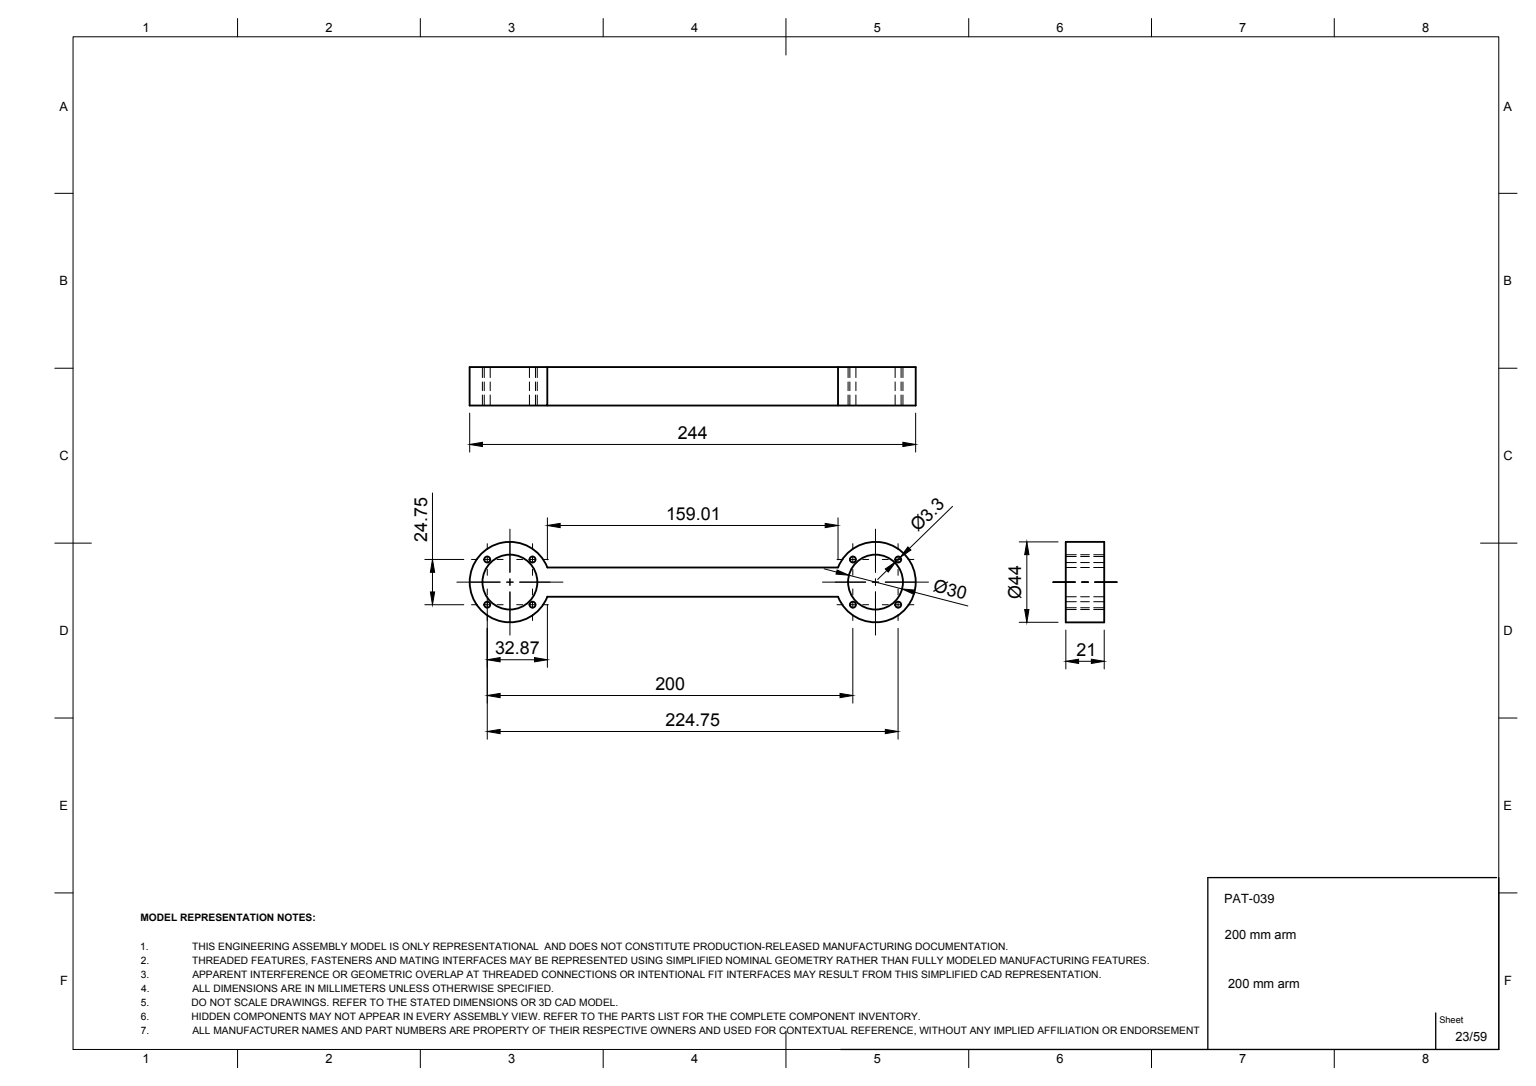
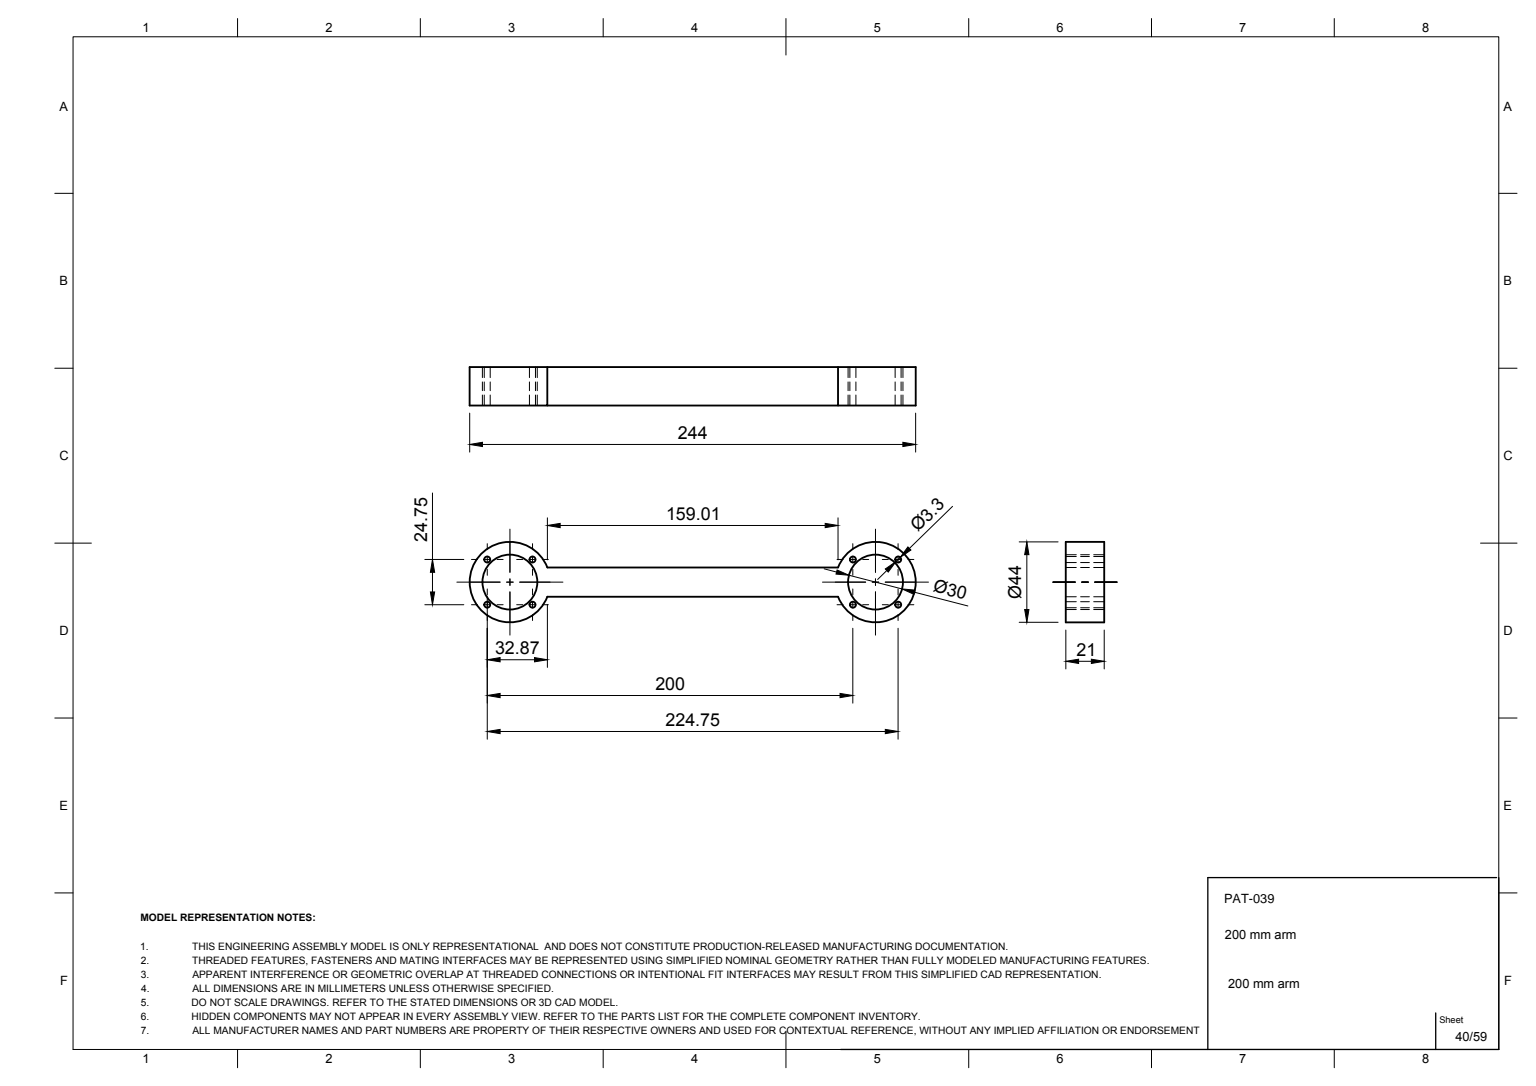
ISO-10303-21;
HEADER;
/* Generated by software containing ST-Developer
 * from STEP Tools, Inc. (www.steptools.com) 
 */

FILE_DESCRIPTION(
/* description */ ('Four-bar parallelogram arm'),
/* implementation_level */ '2;1');

FILE_NAME(
/* name */ '200 mm arm.step',
/* time_stamp */ '2026-10-28T03:24:55-07:00',
/* author */ (''),
/* organization */ (''),
/* preprocessor_version */ 'ST-DEVELOPER v20.2',
/* originating_system */ 'Autodesk Translation Framework v15.17.0.0',
/* authorisation */ '');

FILE_SCHEMA (('AUTOMOTIVE_DESIGN { 1 0 10303 214 3 1 1 }'));
ENDSEC;

DATA;
#10=MECHANICAL_DESIGN_GEOMETRIC_PRESENTATION_REPRESENTATION('',(#639),#14512);
#539=SHAPE_REPRESENTATION_RELATIONSHIP('SRR','None',#14761,#589);
#589=ADVANCED_BREP_SHAPE_REPRESENTATION('',(#696),#14476);
#639=STYLED_ITEM('',(#15101),#696);
#696=MANIFOLD_SOLID_BREP('Body1',#7344);
#807=FACE_BOUND('',#1846,.T.);
#808=FACE_BOUND('',#1847,.T.);
#809=FACE_BOUND('',#1848,.T.);
#810=FACE_BOUND('',#1849,.T.);
#811=FACE_BOUND('',#1850,.T.);
#812=FACE_BOUND('',#1851,.T.);
#813=FACE_BOUND('',#1852,.T.);
#814=FACE_BOUND('',#1853,.T.);
#815=FACE_BOUND('',#1854,.T.);
#816=FACE_BOUND('',#1855,.T.);
#817=FACE_BOUND('',#1859,.T.);
#818=FACE_BOUND('',#1860,.T.);
#819=FACE_BOUND('',#1861,.T.);
#820=FACE_BOUND('',#1862,.T.);
#821=FACE_BOUND('',#1863,.T.);
#822=FACE_BOUND('',#1864,.T.);
#823=FACE_BOUND('',#1865,.T.);
#824=FACE_BOUND('',#1866,.T.);
#825=FACE_BOUND('',#1867,.T.);
#826=FACE_BOUND('',#1868,.T.);
#1089=PLANE('',#8243);
#1090=PLANE('',#8244);
#1091=PLANE('',#8246);
#1092=PLANE('',#8249);
#1341=FACE_OUTER_BOUND('',#1833,.T.);
#1342=FACE_OUTER_BOUND('',#1834,.T.);
#1343=FACE_OUTER_BOUND('',#1835,.T.);
#1344=FACE_OUTER_BOUND('',#1836,.T.);
#1345=FACE_OUTER_BOUND('',#1837,.T.);
#1346=FACE_OUTER_BOUND('',#1838,.T.);
#1347=FACE_OUTER_BOUND('',#1839,.T.);
#1348=FACE_OUTER_BOUND('',#1840,.T.);
#1349=FACE_OUTER_BOUND('',#1841,.T.);
#1350=FACE_OUTER_BOUND('',#1842,.T.);
#1351=FACE_OUTER_BOUND('',#1843,.T.);
#1352=FACE_OUTER_BOUND('',#1844,.T.);
#1353=FACE_OUTER_BOUND('',#1845,.T.);
#1354=FACE_OUTER_BOUND('',#1856,.T.);
#1355=FACE_OUTER_BOUND('',#1857,.T.);
#1356=FACE_OUTER_BOUND('',#1858,.T.);
#1833=EDGE_LOOP('',(#5550,#5551,#5552,#5553));
#1834=EDGE_LOOP('',(#5554,#5555,#5556,#5557));
#1835=EDGE_LOOP('',(#5558,#5559,#5560,#5561));
#1836=EDGE_LOOP('',(#5562,#5563,#5564,#5565));
#1837=EDGE_LOOP('',(#5566,#5567,#5568,#5569));
#1838=EDGE_LOOP('',(#5570,#5571,#5572,#5573));
#1839=EDGE_LOOP('',(#5574,#5575,#5576,#5577));
#1840=EDGE_LOOP('',(#5578,#5579,#5580,#5581));
#1841=EDGE_LOOP('',(#5582,#5583,#5584,#5585));
#1842=EDGE_LOOP('',(#5586,#5587,#5588,#5589));
#1843=EDGE_LOOP('',(#5590,#5591,#5592,#5593));
#1844=EDGE_LOOP('',(#5594,#5595,#5596,#5597));
#1845=EDGE_LOOP('',(#5598,#5599,#5600,#5601));
#1846=EDGE_LOOP('',(#5602));
#1847=EDGE_LOOP('',(#5603));
#1848=EDGE_LOOP('',(#5604));
#1849=EDGE_LOOP('',(#5605));
#1850=EDGE_LOOP('',(#5606));
#1851=EDGE_LOOP('',(#5607));
#1852=EDGE_LOOP('',(#5608));
#1853=EDGE_LOOP('',(#5609));
#1854=EDGE_LOOP('',(#5610));
#1855=EDGE_LOOP('',(#5611));
#1856=EDGE_LOOP('',(#5612,#5613,#5614,#5615));
#1857=EDGE_LOOP('',(#5616,#5617,#5618,#5619));
#1858=EDGE_LOOP('',(#5620,#5621,#5622,#5623));
#1859=EDGE_LOOP('',(#5624));
#1860=EDGE_LOOP('',(#5625));
#1861=EDGE_LOOP('',(#5626));
#1862=EDGE_LOOP('',(#5627));
#1863=EDGE_LOOP('',(#5628));
#1864=EDGE_LOOP('',(#5629));
#1865=EDGE_LOOP('',(#5630));
#1866=EDGE_LOOP('',(#5631));
#1867=EDGE_LOOP('',(#5632));
#1868=EDGE_LOOP('',(#5633));
#2475=LINE('',#12661,#2869);
#2476=LINE('',#12667,#2870);
#2477=LINE('',#12673,#2871);
#2478=LINE('',#12679,#2872);
#2479=LINE('',#12685,#2873);
#2480=LINE('',#12691,#2874);
#2481=LINE('',#12697,#2875);
#2482=LINE('',#12703,#2876);
#2483=LINE('',#12709,#2877);
#2484=LINE('',#12715,#2878);
#2485=LINE('',#12720,#2879);
#2486=LINE('',#12724,#2880);
#2487=LINE('',#12728,#2881);
#2488=LINE('',#12730,#2882);
#2489=LINE('',#12731,#2883);
#2490=LINE('',#12734,#2884);
#2491=LINE('',#12738,#2885);
#2492=LINE('',#12739,#2886);
#2869=VECTOR('',#9681,0.164999999999999);
#2870=VECTOR('',#9688,0.164999999999999);
#2871=VECTOR('',#9695,0.164999999999999);
#2872=VECTOR('',#9702,0.164999999999999);
#2873=VECTOR('',#9709,0.165);
#2874=VECTOR('',#9716,0.165);
#2875=VECTOR('',#9723,0.165);
#2876=VECTOR('',#9730,0.165);
#2877=VECTOR('',#9737,1.5);
#2878=VECTOR('',#9744,1.5);
#2879=VECTOR('',#9749,1.);
#2880=VECTOR('',#9752,1.);
#2881=VECTOR('',#9757,1.);
#2882=VECTOR('',#9758,1.);
#2883=VECTOR('',#9759,1.);
#2884=VECTOR('',#9762,1.);
#2885=VECTOR('',#9767,1.);
#2886=VECTOR('',#9768,1.);
#3212=CIRCLE('',#8211,0.164999999999999);
#3213=CIRCLE('',#8212,0.164999999999999);
#3214=CIRCLE('',#8214,0.164999999999999);
#3215=CIRCLE('',#8215,0.164999999999999);
#3216=CIRCLE('',#8217,0.164999999999999);
#3217=CIRCLE('',#8218,0.164999999999999);
#3218=CIRCLE('',#8220,0.164999999999999);
#3219=CIRCLE('',#8221,0.164999999999999);
#3220=CIRCLE('',#8223,0.165);
#3221=CIRCLE('',#8224,0.165);
#3222=CIRCLE('',#8226,0.165);
#3223=CIRCLE('',#8227,0.165);
#3224=CIRCLE('',#8229,0.165);
#3225=CIRCLE('',#8230,0.165);
#3226=CIRCLE('',#8232,0.165);
#3227=CIRCLE('',#8233,0.165);
#3228=CIRCLE('',#8235,1.5);
#3229=CIRCLE('',#8236,1.5);
#3230=CIRCLE('',#8238,1.5);
#3231=CIRCLE('',#8239,1.5);
#3232=CIRCLE('',#8241,2.2);
#3233=CIRCLE('',#8242,2.2);
#3234=CIRCLE('',#8245,2.2);
#3235=CIRCLE('',#8248,2.2);
#3730=VERTEX_POINT('',#12658);
#3731=VERTEX_POINT('',#12660);
#3732=VERTEX_POINT('',#12664);
#3733=VERTEX_POINT('',#12666);
#3734=VERTEX_POINT('',#12670);
#3735=VERTEX_POINT('',#12672);
#3736=VERTEX_POINT('',#12676);
#3737=VERTEX_POINT('',#12678);
#3738=VERTEX_POINT('',#12682);
#3739=VERTEX_POINT('',#12684);
#3740=VERTEX_POINT('',#12688);
#3741=VERTEX_POINT('',#12690);
#3742=VERTEX_POINT('',#12694);
#3743=VERTEX_POINT('',#12696);
#3744=VERTEX_POINT('',#12700);
#3745=VERTEX_POINT('',#12702);
#3746=VERTEX_POINT('',#12706);
#3747=VERTEX_POINT('',#12708);
#3748=VERTEX_POINT('',#12712);
#3749=VERTEX_POINT('',#12714);
#3750=VERTEX_POINT('',#12718);
#3751=VERTEX_POINT('',#12719);
#3752=VERTEX_POINT('',#12721);
#3753=VERTEX_POINT('',#12723);
#3754=VERTEX_POINT('',#12727);
#3755=VERTEX_POINT('',#12729);
#3756=VERTEX_POINT('',#12733);
#3757=VERTEX_POINT('',#12737);
#4406=EDGE_CURVE('',#3730,#3730,#3212,.T.);
#4407=EDGE_CURVE('',#3730,#3731,#2475,.T.);
#4408=EDGE_CURVE('',#3731,#3731,#3213,.T.);
#4409=EDGE_CURVE('',#3732,#3732,#3214,.T.);
#4410=EDGE_CURVE('',#3732,#3733,#2476,.T.);
#4411=EDGE_CURVE('',#3733,#3733,#3215,.T.);
#4412=EDGE_CURVE('',#3734,#3734,#3216,.T.);
#4413=EDGE_CURVE('',#3734,#3735,#2477,.T.);
#4414=EDGE_CURVE('',#3735,#3735,#3217,.T.);
#4415=EDGE_CURVE('',#3736,#3736,#3218,.T.);
#4416=EDGE_CURVE('',#3736,#3737,#2478,.T.);
#4417=EDGE_CURVE('',#3737,#3737,#3219,.T.);
#4418=EDGE_CURVE('',#3738,#3738,#3220,.T.);
#4419=EDGE_CURVE('',#3738,#3739,#2479,.T.);
#4420=EDGE_CURVE('',#3739,#3739,#3221,.T.);
#4421=EDGE_CURVE('',#3740,#3740,#3222,.T.);
#4422=EDGE_CURVE('',#3740,#3741,#2480,.T.);
#4423=EDGE_CURVE('',#3741,#3741,#3223,.T.);
#4424=EDGE_CURVE('',#3742,#3742,#3224,.T.);
#4425=EDGE_CURVE('',#3742,#3743,#2481,.T.);
#4426=EDGE_CURVE('',#3743,#3743,#3225,.T.);
#4427=EDGE_CURVE('',#3744,#3744,#3226,.T.);
#4428=EDGE_CURVE('',#3744,#3745,#2482,.T.);
#4429=EDGE_CURVE('',#3745,#3745,#3227,.T.);
#4430=EDGE_CURVE('',#3746,#3746,#3228,.T.);
#4431=EDGE_CURVE('',#3746,#3747,#2483,.T.);
#4432=EDGE_CURVE('',#3747,#3747,#3229,.T.);
#4433=EDGE_CURVE('',#3748,#3748,#3230,.T.);
#4434=EDGE_CURVE('',#3748,#3749,#2484,.T.);
#4435=EDGE_CURVE('',#3749,#3749,#3231,.T.);
#4436=EDGE_CURVE('',#3750,#3751,#2485,.T.);
#4437=EDGE_CURVE('',#3752,#3750,#3232,.T.);
#4438=EDGE_CURVE('',#3753,#3752,#2486,.T.);
#4439=EDGE_CURVE('',#3753,#3751,#3233,.T.);
#4440=EDGE_CURVE('',#3754,#3751,#2487,.T.);
#4441=EDGE_CURVE('',#3755,#3754,#2488,.T.);
#4442=EDGE_CURVE('',#3750,#3755,#2489,.T.);
#4443=EDGE_CURVE('',#3753,#3756,#2490,.T.);
#4444=EDGE_CURVE('',#3754,#3756,#3234,.T.);
#4445=EDGE_CURVE('',#3757,#3752,#2491,.T.);
#4446=EDGE_CURVE('',#3756,#3757,#2492,.T.);
#4447=EDGE_CURVE('',#3755,#3757,#3235,.T.);
#5550=ORIENTED_EDGE('',*,*,#4406,.F.);
#5551=ORIENTED_EDGE('',*,*,#4407,.T.);
#5552=ORIENTED_EDGE('',*,*,#4408,.F.);
#5553=ORIENTED_EDGE('',*,*,#4407,.F.);
#5554=ORIENTED_EDGE('',*,*,#4409,.F.);
#5555=ORIENTED_EDGE('',*,*,#4410,.T.);
#5556=ORIENTED_EDGE('',*,*,#4411,.F.);
#5557=ORIENTED_EDGE('',*,*,#4410,.F.);
#5558=ORIENTED_EDGE('',*,*,#4412,.F.);
#5559=ORIENTED_EDGE('',*,*,#4413,.T.);
#5560=ORIENTED_EDGE('',*,*,#4414,.F.);
#5561=ORIENTED_EDGE('',*,*,#4413,.F.);
#5562=ORIENTED_EDGE('',*,*,#4415,.F.);
#5563=ORIENTED_EDGE('',*,*,#4416,.T.);
#5564=ORIENTED_EDGE('',*,*,#4417,.F.);
#5565=ORIENTED_EDGE('',*,*,#4416,.F.);
#5566=ORIENTED_EDGE('',*,*,#4418,.F.);
#5567=ORIENTED_EDGE('',*,*,#4419,.T.);
#5568=ORIENTED_EDGE('',*,*,#4420,.F.);
#5569=ORIENTED_EDGE('',*,*,#4419,.F.);
#5570=ORIENTED_EDGE('',*,*,#4421,.F.);
#5571=ORIENTED_EDGE('',*,*,#4422,.T.);
#5572=ORIENTED_EDGE('',*,*,#4423,.F.);
#5573=ORIENTED_EDGE('',*,*,#4422,.F.);
#5574=ORIENTED_EDGE('',*,*,#4424,.F.);
#5575=ORIENTED_EDGE('',*,*,#4425,.T.);
#5576=ORIENTED_EDGE('',*,*,#4426,.F.);
#5577=ORIENTED_EDGE('',*,*,#4425,.F.);
#5578=ORIENTED_EDGE('',*,*,#4427,.F.);
#5579=ORIENTED_EDGE('',*,*,#4428,.T.);
#5580=ORIENTED_EDGE('',*,*,#4429,.F.);
#5581=ORIENTED_EDGE('',*,*,#4428,.F.);
#5582=ORIENTED_EDGE('',*,*,#4430,.F.);
#5583=ORIENTED_EDGE('',*,*,#4431,.T.);
#5584=ORIENTED_EDGE('',*,*,#4432,.F.);
#5585=ORIENTED_EDGE('',*,*,#4431,.F.);
#5586=ORIENTED_EDGE('',*,*,#4433,.F.);
#5587=ORIENTED_EDGE('',*,*,#4434,.T.);
#5588=ORIENTED_EDGE('',*,*,#4435,.F.);
#5589=ORIENTED_EDGE('',*,*,#4434,.F.);
#5590=ORIENTED_EDGE('',*,*,#4436,.F.);
#5591=ORIENTED_EDGE('',*,*,#4437,.F.);
#5592=ORIENTED_EDGE('',*,*,#4438,.F.);
#5593=ORIENTED_EDGE('',*,*,#4439,.T.);
#5594=ORIENTED_EDGE('',*,*,#4436,.T.);
#5595=ORIENTED_EDGE('',*,*,#4440,.F.);
#5596=ORIENTED_EDGE('',*,*,#4441,.F.);
#5597=ORIENTED_EDGE('',*,*,#4442,.F.);
#5598=ORIENTED_EDGE('',*,*,#4439,.F.);
#5599=ORIENTED_EDGE('',*,*,#4443,.T.);
#5600=ORIENTED_EDGE('',*,*,#4444,.F.);
#5601=ORIENTED_EDGE('',*,*,#4440,.T.);
#5602=ORIENTED_EDGE('',*,*,#4418,.T.);
#5603=ORIENTED_EDGE('',*,*,#4421,.T.);
#5604=ORIENTED_EDGE('',*,*,#4424,.T.);
#5605=ORIENTED_EDGE('',*,*,#4427,.T.);
#5606=ORIENTED_EDGE('',*,*,#4430,.T.);
#5607=ORIENTED_EDGE('',*,*,#4433,.T.);
#5608=ORIENTED_EDGE('',*,*,#4415,.T.);
#5609=ORIENTED_EDGE('',*,*,#4412,.T.);
#5610=ORIENTED_EDGE('',*,*,#4409,.T.);
#5611=ORIENTED_EDGE('',*,*,#4406,.T.);
#5612=ORIENTED_EDGE('',*,*,#4438,.T.);
#5613=ORIENTED_EDGE('',*,*,#4445,.F.);
#5614=ORIENTED_EDGE('',*,*,#4446,.F.);
#5615=ORIENTED_EDGE('',*,*,#4443,.F.);
#5616=ORIENTED_EDGE('',*,*,#4441,.T.);
#5617=ORIENTED_EDGE('',*,*,#4444,.T.);
#5618=ORIENTED_EDGE('',*,*,#4446,.T.);
#5619=ORIENTED_EDGE('',*,*,#4447,.F.);
#5620=ORIENTED_EDGE('',*,*,#4442,.T.);
#5621=ORIENTED_EDGE('',*,*,#4447,.T.);
#5622=ORIENTED_EDGE('',*,*,#4445,.T.);
#5623=ORIENTED_EDGE('',*,*,#4437,.T.);
#5624=ORIENTED_EDGE('',*,*,#4420,.T.);
#5625=ORIENTED_EDGE('',*,*,#4423,.T.);
#5626=ORIENTED_EDGE('',*,*,#4426,.T.);
#5627=ORIENTED_EDGE('',*,*,#4429,.T.);
#5628=ORIENTED_EDGE('',*,*,#4432,.T.);
#5629=ORIENTED_EDGE('',*,*,#4435,.T.);
#5630=ORIENTED_EDGE('',*,*,#4417,.T.);
#5631=ORIENTED_EDGE('',*,*,#4414,.T.);
#5632=ORIENTED_EDGE('',*,*,#4411,.T.);
#5633=ORIENTED_EDGE('',*,*,#4408,.T.);
#6767=CYLINDRICAL_SURFACE('',#8210,0.164999999999999);
#6768=CYLINDRICAL_SURFACE('',#8213,0.164999999999999);
#6769=CYLINDRICAL_SURFACE('',#8216,0.164999999999999);
#6770=CYLINDRICAL_SURFACE('',#8219,0.164999999999999);
#6771=CYLINDRICAL_SURFACE('',#8222,0.165);
#6772=CYLINDRICAL_SURFACE('',#8225,0.165);
#6773=CYLINDRICAL_SURFACE('',#8228,0.165);
#6774=CYLINDRICAL_SURFACE('',#8231,0.165);
#6775=CYLINDRICAL_SURFACE('',#8234,1.5);
#6776=CYLINDRICAL_SURFACE('',#8237,1.5);
#6777=CYLINDRICAL_SURFACE('',#8240,2.2);
#6778=CYLINDRICAL_SURFACE('',#8247,2.2);
#7046=ADVANCED_FACE('',(#1341),#6767,.F.);
#7047=ADVANCED_FACE('',(#1342),#6768,.F.);
#7048=ADVANCED_FACE('',(#1343),#6769,.F.);
#7049=ADVANCED_FACE('',(#1344),#6770,.F.);
#7050=ADVANCED_FACE('',(#1345),#6771,.F.);
#7051=ADVANCED_FACE('',(#1346),#6772,.F.);
#7052=ADVANCED_FACE('',(#1347),#6773,.F.);
#7053=ADVANCED_FACE('',(#1348),#6774,.F.);
#7054=ADVANCED_FACE('',(#1349),#6775,.F.);
#7055=ADVANCED_FACE('',(#1350),#6776,.F.);
#7056=ADVANCED_FACE('',(#1351),#6777,.T.);
#7057=ADVANCED_FACE('',(#1352),#1089,.T.);
#7058=ADVANCED_FACE('',(#1353,#807,#808,#809,#810,#811,#812,#813,#814,#815,
#816),#1090,.F.);
#7059=ADVANCED_FACE('',(#1354),#1091,.T.);
#7060=ADVANCED_FACE('',(#1355),#6778,.T.);
#7061=ADVANCED_FACE('',(#1356,#817,#818,#819,#820,#821,#822,#823,#824,#825,
#826),#1092,.T.);
#7344=CLOSED_SHELL('',(#7046,#7047,#7048,#7049,#7050,#7051,#7052,#7053,
#7054,#7055,#7056,#7057,#7058,#7059,#7060,#7061));
#8209=AXIS2_PLACEMENT_3D('',#12656,#9675,#9676);
#8210=AXIS2_PLACEMENT_3D('',#12657,#9677,#9678);
#8211=AXIS2_PLACEMENT_3D('',#12659,#9679,#9680);
#8212=AXIS2_PLACEMENT_3D('',#12662,#9682,#9683);
#8213=AXIS2_PLACEMENT_3D('',#12663,#9684,#9685);
#8214=AXIS2_PLACEMENT_3D('',#12665,#9686,#9687);
#8215=AXIS2_PLACEMENT_3D('',#12668,#9689,#9690);
#8216=AXIS2_PLACEMENT_3D('',#12669,#9691,#9692);
#8217=AXIS2_PLACEMENT_3D('',#12671,#9693,#9694);
#8218=AXIS2_PLACEMENT_3D('',#12674,#9696,#9697);
#8219=AXIS2_PLACEMENT_3D('',#12675,#9698,#9699);
#8220=AXIS2_PLACEMENT_3D('',#12677,#9700,#9701);
#8221=AXIS2_PLACEMENT_3D('',#12680,#9703,#9704);
#8222=AXIS2_PLACEMENT_3D('',#12681,#9705,#9706);
#8223=AXIS2_PLACEMENT_3D('',#12683,#9707,#9708);
#8224=AXIS2_PLACEMENT_3D('',#12686,#9710,#9711);
#8225=AXIS2_PLACEMENT_3D('',#12687,#9712,#9713);
#8226=AXIS2_PLACEMENT_3D('',#12689,#9714,#9715);
#8227=AXIS2_PLACEMENT_3D('',#12692,#9717,#9718);
#8228=AXIS2_PLACEMENT_3D('',#12693,#9719,#9720);
#8229=AXIS2_PLACEMENT_3D('',#12695,#9721,#9722);
#8230=AXIS2_PLACEMENT_3D('',#12698,#9724,#9725);
#8231=AXIS2_PLACEMENT_3D('',#12699,#9726,#9727);
#8232=AXIS2_PLACEMENT_3D('',#12701,#9728,#9729);
#8233=AXIS2_PLACEMENT_3D('',#12704,#9731,#9732);
#8234=AXIS2_PLACEMENT_3D('',#12705,#9733,#9734);
#8235=AXIS2_PLACEMENT_3D('',#12707,#9735,#9736);
#8236=AXIS2_PLACEMENT_3D('',#12710,#9738,#9739);
#8237=AXIS2_PLACEMENT_3D('',#12711,#9740,#9741);
#8238=AXIS2_PLACEMENT_3D('',#12713,#9742,#9743);
#8239=AXIS2_PLACEMENT_3D('',#12716,#9745,#9746);
#8240=AXIS2_PLACEMENT_3D('',#12717,#9747,#9748);
#8241=AXIS2_PLACEMENT_3D('',#12722,#9750,#9751);
#8242=AXIS2_PLACEMENT_3D('',#12725,#9753,#9754);
#8243=AXIS2_PLACEMENT_3D('',#12726,#9755,#9756);
#8244=AXIS2_PLACEMENT_3D('',#12732,#9760,#9761);
#8245=AXIS2_PLACEMENT_3D('',#12735,#9763,#9764);
#8246=AXIS2_PLACEMENT_3D('',#12736,#9765,#9766);
#8247=AXIS2_PLACEMENT_3D('',#12740,#9769,#9770);
#8248=AXIS2_PLACEMENT_3D('',#12741,#9771,#9772);
#8249=AXIS2_PLACEMENT_3D('',#12742,#9773,#9774);
#9675=DIRECTION('axis',(0.,0.,1.));
#9676=DIRECTION('refdir',(1.,0.,0.));
#9677=DIRECTION('center_axis',(0.,1.,0.));
#9678=DIRECTION('ref_axis',(1.,0.,0.));
#9679=DIRECTION('center_axis',(0.,1.,0.));
#9680=DIRECTION('ref_axis',(1.,0.,0.));
#9681=DIRECTION('',(0.,1.,0.));
#9682=DIRECTION('center_axis',(0.,-1.,0.));
#9683=DIRECTION('ref_axis',(1.,0.,0.));
#9684=DIRECTION('center_axis',(0.,1.,0.));
#9685=DIRECTION('ref_axis',(1.,0.,0.));
#9686=DIRECTION('center_axis',(0.,1.,0.));
#9687=DIRECTION('ref_axis',(1.,0.,0.));
#9688=DIRECTION('',(0.,1.,0.));
#9689=DIRECTION('center_axis',(0.,-1.,0.));
#9690=DIRECTION('ref_axis',(1.,0.,0.));
#9691=DIRECTION('center_axis',(0.,1.,0.));
#9692=DIRECTION('ref_axis',(1.,0.,0.));
#9693=DIRECTION('center_axis',(0.,1.,0.));
#9694=DIRECTION('ref_axis',(1.,0.,0.));
#9695=DIRECTION('',(0.,1.,0.));
#9696=DIRECTION('center_axis',(0.,-1.,0.));
#9697=DIRECTION('ref_axis',(1.,0.,0.));
#9698=DIRECTION('center_axis',(0.,1.,0.));
#9699=DIRECTION('ref_axis',(1.,0.,0.));
#9700=DIRECTION('center_axis',(0.,1.,0.));
#9701=DIRECTION('ref_axis',(1.,0.,0.));
#9702=DIRECTION('',(0.,1.,0.));
#9703=DIRECTION('center_axis',(0.,-1.,0.));
#9704=DIRECTION('ref_axis',(1.,0.,0.));
#9705=DIRECTION('center_axis',(0.,1.,0.));
#9706=DIRECTION('ref_axis',(1.,0.,0.));
#9707=DIRECTION('center_axis',(0.,1.,0.));
#9708=DIRECTION('ref_axis',(1.,0.,0.));
#9709=DIRECTION('',(0.,1.,0.));
#9710=DIRECTION('center_axis',(0.,-1.,0.));
#9711=DIRECTION('ref_axis',(1.,0.,0.));
#9712=DIRECTION('center_axis',(0.,1.,0.));
#9713=DIRECTION('ref_axis',(1.,0.,0.));
#9714=DIRECTION('center_axis',(0.,1.,0.));
#9715=DIRECTION('ref_axis',(1.,0.,0.));
#9716=DIRECTION('',(0.,1.,0.));
#9717=DIRECTION('center_axis',(0.,-1.,0.));
#9718=DIRECTION('ref_axis',(1.,0.,0.));
#9719=DIRECTION('center_axis',(0.,1.,0.));
#9720=DIRECTION('ref_axis',(1.,0.,0.));
#9721=DIRECTION('center_axis',(0.,1.,0.));
#9722=DIRECTION('ref_axis',(1.,0.,0.));
#9723=DIRECTION('',(0.,1.,0.));
#9724=DIRECTION('center_axis',(0.,-1.,0.));
#9725=DIRECTION('ref_axis',(1.,0.,0.));
#9726=DIRECTION('center_axis',(0.,1.,0.));
#9727=DIRECTION('ref_axis',(1.,0.,0.));
#9728=DIRECTION('center_axis',(0.,1.,0.));
#9729=DIRECTION('ref_axis',(1.,0.,0.));
#9730=DIRECTION('',(0.,1.,0.));
#9731=DIRECTION('center_axis',(0.,-1.,0.));
#9732=DIRECTION('ref_axis',(1.,0.,0.));
#9733=DIRECTION('center_axis',(0.,1.,0.));
#9734=DIRECTION('ref_axis',(1.,0.,0.));
#9735=DIRECTION('center_axis',(0.,1.,0.));
#9736=DIRECTION('ref_axis',(1.,0.,0.));
#9737=DIRECTION('',(0.,1.,0.));
#9738=DIRECTION('center_axis',(0.,-1.,0.));
#9739=DIRECTION('ref_axis',(1.,0.,0.));
#9740=DIRECTION('center_axis',(0.,1.,0.));
#9741=DIRECTION('ref_axis',(1.,0.,0.));
#9742=DIRECTION('center_axis',(0.,1.,0.));
#9743=DIRECTION('ref_axis',(1.,0.,0.));
#9744=DIRECTION('',(0.,1.,0.));
#9745=DIRECTION('center_axis',(0.,-1.,0.));
#9746=DIRECTION('ref_axis',(1.,0.,0.));
#9747=DIRECTION('center_axis',(0.,1.,0.));
#9748=DIRECTION('ref_axis',(1.,0.,0.));
#9749=DIRECTION('',(0.,-1.,0.));
#9750=DIRECTION('center_axis',(0.,1.,0.));
#9751=DIRECTION('ref_axis',(1.,0.,0.));
#9752=DIRECTION('',(0.,1.,0.));
#9753=DIRECTION('center_axis',(0.,1.,0.));
#9754=DIRECTION('ref_axis',(1.,0.,0.));
#9755=DIRECTION('center_axis',(0.,0.,-1.));
#9756=DIRECTION('ref_axis',(-1.,0.,0.));
#9757=DIRECTION('',(1.,0.,0.));
#9758=DIRECTION('',(0.,-1.,0.));
#9759=DIRECTION('',(-1.,0.,0.));
#9760=DIRECTION('center_axis',(0.,1.,0.));
#9761=DIRECTION('ref_axis',(1.,0.,0.));
#9762=DIRECTION('',(-1.,0.,0.));
#9763=DIRECTION('center_axis',(0.,1.,0.));
#9764=DIRECTION('ref_axis',(1.,0.,0.));
#9765=DIRECTION('center_axis',(0.,0.,1.));
#9766=DIRECTION('ref_axis',(1.,0.,0.));
#9767=DIRECTION('',(1.,0.,0.));
#9768=DIRECTION('',(0.,1.,0.));
#9769=DIRECTION('center_axis',(0.,1.,0.));
#9770=DIRECTION('ref_axis',(-1.,0.,-1.22464679914735E-16));
#9771=DIRECTION('center_axis',(0.,1.,0.));
#9772=DIRECTION('ref_axis',(1.,0.,0.));
#9773=DIRECTION('center_axis',(0.,1.,0.));
#9774=DIRECTION('ref_axis',(1.,0.,0.));
#12656=CARTESIAN_POINT('',(0.,0.,0.));
#12657=CARTESIAN_POINT('Origin',(18.7625631329235,-1.15,6.76256313292354));
#12658=CARTESIAN_POINT('',(18.5975631329235,-1.05,6.76256313292354));
#12659=CARTESIAN_POINT('Origin',(18.7625631329235,-1.05,6.76256313292354));
#12660=CARTESIAN_POINT('',(18.5975631329235,1.05,6.76256313292354));
#12661=CARTESIAN_POINT('',(18.5975631329235,-1.15,6.76256313292354));
#12662=CARTESIAN_POINT('Origin',(18.7625631329235,1.05,6.76256313292354));
#12663=CARTESIAN_POINT('Origin',(18.7625631329235,-1.15,9.23743686707646));
#12664=CARTESIAN_POINT('',(18.5975631329235,-1.05,9.23743686707646));
#12665=CARTESIAN_POINT('Origin',(18.7625631329235,-1.05,9.23743686707646));
#12666=CARTESIAN_POINT('',(18.5975631329235,1.05,9.23743686707646));
#12667=CARTESIAN_POINT('',(18.5975631329235,-1.15,9.23743686707646));
#12668=CARTESIAN_POINT('Origin',(18.7625631329235,1.05,9.23743686707646));
#12669=CARTESIAN_POINT('Origin',(21.2374368670765,-1.15,9.23743686707646));
#12670=CARTESIAN_POINT('',(21.0724368670765,-1.05,9.23743686707646));
#12671=CARTESIAN_POINT('Origin',(21.2374368670765,-1.05,9.23743686707646));
#12672=CARTESIAN_POINT('',(21.0724368670765,1.05,9.23743686707646));
#12673=CARTESIAN_POINT('',(21.0724368670765,-1.15,9.23743686707646));
#12674=CARTESIAN_POINT('Origin',(21.2374368670765,1.05,9.23743686707646));
#12675=CARTESIAN_POINT('Origin',(21.2374368670765,-1.15,6.76256313292354));
#12676=CARTESIAN_POINT('',(21.0724368670765,-1.05,6.76256313292354));
#12677=CARTESIAN_POINT('Origin',(21.2374368670765,-1.05,6.76256313292354));
#12678=CARTESIAN_POINT('',(21.0724368670765,1.05,6.76256313292354));
#12679=CARTESIAN_POINT('',(21.0724368670765,-1.15,6.76256313292354));
#12680=CARTESIAN_POINT('Origin',(21.2374368670765,1.05,6.76256313292354));
#12681=CARTESIAN_POINT('Origin',(-1.23743686707646,-1.15,6.76256313292354));
#12682=CARTESIAN_POINT('',(-1.40243686707646,-1.05,6.76256313292354));
#12683=CARTESIAN_POINT('Origin',(-1.23743686707646,-1.05,6.76256313292354));
#12684=CARTESIAN_POINT('',(-1.40243686707646,1.05,6.76256313292354));
#12685=CARTESIAN_POINT('',(-1.40243686707646,-1.15,6.76256313292354));
#12686=CARTESIAN_POINT('Origin',(-1.23743686707646,1.05,6.76256313292354));
#12687=CARTESIAN_POINT('Origin',(-1.23743686707646,-1.15,9.23743686707646));
#12688=CARTESIAN_POINT('',(-1.40243686707646,-1.05,9.23743686707646));
#12689=CARTESIAN_POINT('Origin',(-1.23743686707646,-1.05,9.23743686707646));
#12690=CARTESIAN_POINT('',(-1.40243686707646,1.05,9.23743686707646));
#12691=CARTESIAN_POINT('',(-1.40243686707646,-1.15,9.23743686707646));
#12692=CARTESIAN_POINT('Origin',(-1.23743686707646,1.05,9.23743686707646));
#12693=CARTESIAN_POINT('Origin',(1.23743686707646,-1.15,9.23743686707646));
#12694=CARTESIAN_POINT('',(1.07243686707646,-1.05,9.23743686707646));
#12695=CARTESIAN_POINT('Origin',(1.23743686707646,-1.05,9.23743686707646));
#12696=CARTESIAN_POINT('',(1.07243686707646,1.05,9.23743686707646));
#12697=CARTESIAN_POINT('',(1.07243686707646,-1.15,9.23743686707646));
#12698=CARTESIAN_POINT('Origin',(1.23743686707646,1.05,9.23743686707646));
#12699=CARTESIAN_POINT('Origin',(1.23743686707646,-1.15,6.76256313292354));
#12700=CARTESIAN_POINT('',(1.07243686707646,-1.05,6.76256313292354));
#12701=CARTESIAN_POINT('Origin',(1.23743686707646,-1.05,6.76256313292354));
#12702=CARTESIAN_POINT('',(1.07243686707646,1.05,6.76256313292354));
#12703=CARTESIAN_POINT('',(1.07243686707646,-1.15,6.76256313292354));
#12704=CARTESIAN_POINT('Origin',(1.23743686707646,1.05,6.76256313292354));
#12705=CARTESIAN_POINT('Origin',(0.,-1.15,8.));
#12706=CARTESIAN_POINT('',(-1.5,-1.05,8.));
#12707=CARTESIAN_POINT('Origin',(0.,-1.05,8.));
#12708=CARTESIAN_POINT('',(-1.5,1.05,8.));
#12709=CARTESIAN_POINT('',(-1.5,-1.15,8.));
#12710=CARTESIAN_POINT('Origin',(0.,1.05,8.));
#12711=CARTESIAN_POINT('Origin',(20.,-1.15,8.));
#12712=CARTESIAN_POINT('',(18.5,-1.05,8.));
#12713=CARTESIAN_POINT('Origin',(20.,-1.05,8.));
#12714=CARTESIAN_POINT('',(18.5,1.05,8.));
#12715=CARTESIAN_POINT('',(18.5,-1.15,8.));
#12716=CARTESIAN_POINT('Origin',(20.,1.05,8.));
#12717=CARTESIAN_POINT('Origin',(20.,-1.05,8.));
#12718=CARTESIAN_POINT('',(17.9506098468081,1.05,7.2));
#12719=CARTESIAN_POINT('',(17.9506098468081,-1.05,7.2));
#12720=CARTESIAN_POINT('',(17.9506098468081,-1.05,7.2));
#12721=CARTESIAN_POINT('',(17.9506098468081,1.05,8.8));
#12722=CARTESIAN_POINT('Origin',(20.,1.05,8.));
#12723=CARTESIAN_POINT('',(17.9506098468081,-1.05,8.8));
#12724=CARTESIAN_POINT('',(17.9506098468081,-1.05,8.8));
#12725=CARTESIAN_POINT('Origin',(20.,-1.05,8.));
#12726=CARTESIAN_POINT('Origin',(20.,-1.05,7.2));
#12727=CARTESIAN_POINT('',(2.04939015319192,-1.05,7.2));
#12728=CARTESIAN_POINT('',(0.,-1.05,7.2));
#12729=CARTESIAN_POINT('',(2.04939015319192,1.05,7.2));
#12730=CARTESIAN_POINT('',(2.04939015319192,-1.05,7.2));
#12731=CARTESIAN_POINT('',(0.,1.05,7.2));
#12732=CARTESIAN_POINT('Origin',(0.,-1.05,8.));
#12733=CARTESIAN_POINT('',(2.04939015319192,-1.05,8.8));
#12734=CARTESIAN_POINT('',(20.,-1.05,8.8));
#12735=CARTESIAN_POINT('Origin',(0.,-1.05,8.));
#12736=CARTESIAN_POINT('Origin',(0.,-1.05,8.8));
#12737=CARTESIAN_POINT('',(2.04939015319192,1.05,8.8));
#12738=CARTESIAN_POINT('',(20.,1.05,8.8));
#12739=CARTESIAN_POINT('',(2.04939015319192,-1.05,8.8));
#12740=CARTESIAN_POINT('Origin',(0.,-1.05,8.));
#12741=CARTESIAN_POINT('Origin',(0.,1.05,8.));
#12742=CARTESIAN_POINT('Origin',(0.,1.05,8.));
#14419=UNCERTAINTY_MEASURE_WITH_UNIT(LENGTH_MEASURE(0.001),#14513,
'DISTANCE_ACCURACY_VALUE',
'Maximum model space distance between geometric entities at asserted c
onnectivities');
#14455=UNCERTAINTY_MEASURE_WITH_UNIT(LENGTH_MEASURE(0.001),#14513,
'DISTANCE_ACCURACY_VALUE',
'Maximum model space distance between geometric entities at asserted c
onnectivities');
#14476=(
GEOMETRIC_REPRESENTATION_CONTEXT(3)
GLOBAL_UNCERTAINTY_ASSIGNED_CONTEXT((#14419))
GLOBAL_UNIT_ASSIGNED_CONTEXT((#14513,#14515,#14516))
REPRESENTATION_CONTEXT('','3D')
);
#14512=(
GEOMETRIC_REPRESENTATION_CONTEXT(3)
GLOBAL_UNCERTAINTY_ASSIGNED_CONTEXT((#14455))
GLOBAL_UNIT_ASSIGNED_CONTEXT((#14513,#14515,#14516))
REPRESENTATION_CONTEXT('','3D')
);
#14513=(
LENGTH_UNIT()
NAMED_UNIT(*)
SI_UNIT(.CENTI.,.METRE.)
);
#14515=(
NAMED_UNIT(*)
PLANE_ANGLE_UNIT()
SI_UNIT($,.RADIAN.)
);
#14516=(
NAMED_UNIT(*)
SI_UNIT($,.STERADIAN.)
SOLID_ANGLE_UNIT()
);
#14537=SHAPE_DEFINITION_REPRESENTATION(#14593,#14761);
#14593=PRODUCT_DEFINITION_SHAPE('',$,#14818);
#14761=SHAPE_REPRESENTATION('',(#8209),#14476);
#14797=PRODUCT_DEFINITION_CONTEXT('part definition',#14967,'design');
#14818=PRODUCT_DEFINITION('200 mm arm','200 mm arm',#14874,#14797);
#14874=PRODUCT_DEFINITION_FORMATION('',$,#14989);
#14967=APPLICATION_CONTEXT(
'Core Data for Automotive Mechanical Design Process');
#14968=PRODUCT_CONTEXT('part definition',#14967,'mechanical');
#14989=PRODUCT('200 mm arm','200 mm arm','200 mm arm',(#14968));
#15095=COLOUR_RGB('Off White',0.89,0.88,0.83);
#15096=FILL_AREA_STYLE_COLOUR('',#15095);
#15097=FILL_AREA_STYLE('',(#15096));
#15098=SURFACE_STYLE_FILL_AREA(#15097);
#15099=SURFACE_SIDE_STYLE('',(#15098));
#15100=SURFACE_STYLE_USAGE(.BOTH.,#15099);
#15101=PRESENTATION_STYLE_ASSIGNMENT((#15100));
ENDSEC;
END-ISO-10303-21;
